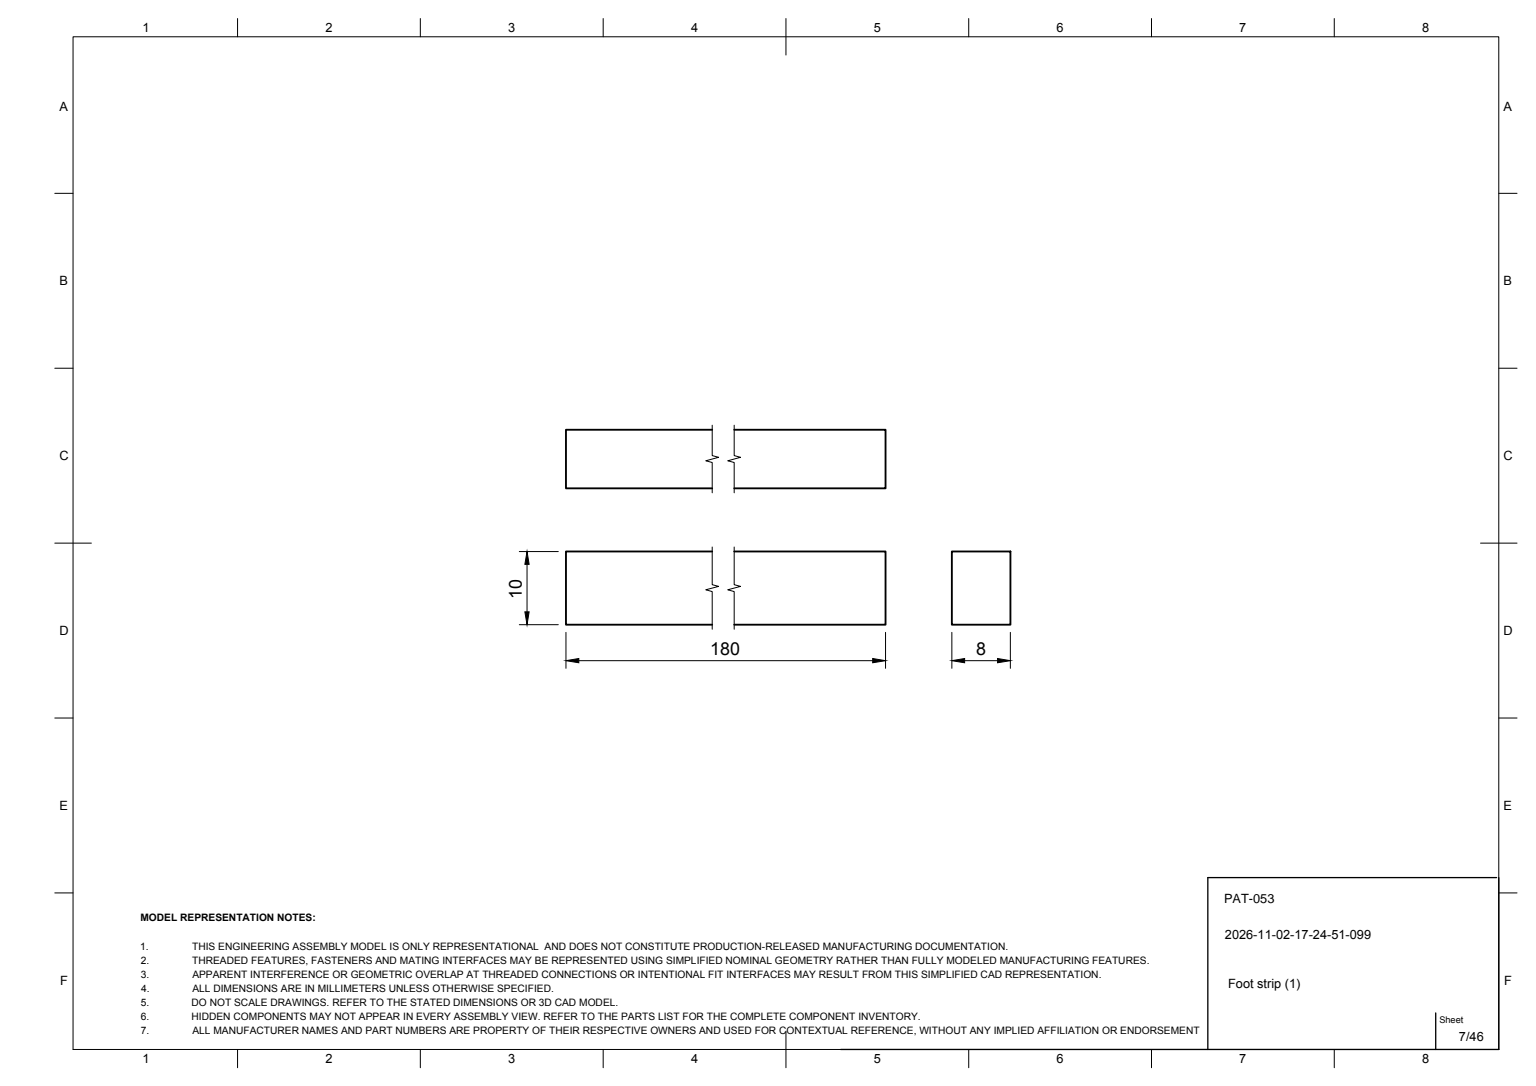
ISO-10303-21;
HEADER;
/* Generated by software containing ST-Developer
 * from STEP Tools, Inc. (www.steptools.com) 
 */

FILE_DESCRIPTION(
/* description */ ('Hand-operated arbor press'),
/* implementation_level */ '2;1');

FILE_NAME(
/* name */ 'Foot strip (1).step',
/* time_stamp */ '2026-10-28T03:25:25-07:00',
/* author */ (''),
/* organization */ (''),
/* preprocessor_version */ 'ST-DEVELOPER v20.2',
/* originating_system */ 'Autodesk Translation Framework v15.17.0.0',
/* authorisation */ '');

FILE_SCHEMA (('AUTOMOTIVE_DESIGN { 1 0 10303 214 3 1 1 }'));
ENDSEC;

DATA;
#10=MECHANICAL_DESIGN_GEOMETRIC_PRESENTATION_REPRESENTATION('',(#588),#32751);
#504=SHAPE_REPRESENTATION_RELATIONSHIP('SRR','None',#32933,#546);
#546=ADVANCED_BREP_SHAPE_REPRESENTATION('',(#637),#32707);
#588=STYLED_ITEM('',(#33228),#637);
#637=MANIFOLD_SOLID_BREP('Body1',#12485);
#861=PLANE('',#13046);
#862=PLANE('',#13047);
#863=PLANE('',#13048);
#864=PLANE('',#13049);
#865=PLANE('',#13050);
#866=PLANE('',#13051);
#1315=FACE_OUTER_BOUND('',#2016,.T.);
#1316=FACE_OUTER_BOUND('',#2017,.T.);
#1317=FACE_OUTER_BOUND('',#2018,.T.);
#1318=FACE_OUTER_BOUND('',#2019,.T.);
#1319=FACE_OUTER_BOUND('',#2020,.T.);
#1320=FACE_OUTER_BOUND('',#2021,.T.);
#2016=EDGE_LOOP('',(#8432,#8433,#8434,#8435));
#2017=EDGE_LOOP('',(#8436,#8437,#8438,#8439));
#2018=EDGE_LOOP('',(#8440,#8441,#8442,#8443));
#2019=EDGE_LOOP('',(#8444,#8445,#8446,#8447));
#2020=EDGE_LOOP('',(#8448,#8449,#8450,#8451));
#2021=EDGE_LOOP('',(#8452,#8453,#8454,#8455));
#2858=LINE('',#17758,#4029);
#2859=LINE('',#17760,#4030);
#2860=LINE('',#17762,#4031);
#2861=LINE('',#17763,#4032);
#2862=LINE('',#17766,#4033);
#2863=LINE('',#17768,#4034);
#2864=LINE('',#17769,#4035);
#2865=LINE('',#17772,#4036);
#2866=LINE('',#17774,#4037);
#2867=LINE('',#17775,#4038);
#2868=LINE('',#17777,#4039);
#2869=LINE('',#17778,#4040);
#4029=VECTOR('',#14285,1.);
#4030=VECTOR('',#14286,1.);
#4031=VECTOR('',#14287,1.);
#4032=VECTOR('',#14288,1.);
#4033=VECTOR('',#14291,1.);
#4034=VECTOR('',#14292,1.);
#4035=VECTOR('',#14293,1.);
#4036=VECTOR('',#14296,1.);
#4037=VECTOR('',#14297,1.);
#4038=VECTOR('',#14298,1.);
#4039=VECTOR('',#14301,1.);
#4040=VECTOR('',#14302,1.);
#5592=VERTEX_POINT('',#17756);
#5593=VERTEX_POINT('',#17757);
#5594=VERTEX_POINT('',#17759);
#5595=VERTEX_POINT('',#17761);
#5596=VERTEX_POINT('',#17765);
#5597=VERTEX_POINT('',#17767);
#5598=VERTEX_POINT('',#17771);
#5599=VERTEX_POINT('',#17773);
#6719=EDGE_CURVE('',#5592,#5593,#2858,.T.);
#6720=EDGE_CURVE('',#5593,#5594,#2859,.T.);
#6721=EDGE_CURVE('',#5595,#5594,#2860,.T.);
#6722=EDGE_CURVE('',#5592,#5595,#2861,.T.);
#6723=EDGE_CURVE('',#5596,#5592,#2862,.T.);
#6724=EDGE_CURVE('',#5597,#5595,#2863,.T.);
#6725=EDGE_CURVE('',#5596,#5597,#2864,.T.);
#6726=EDGE_CURVE('',#5598,#5596,#2865,.T.);
#6727=EDGE_CURVE('',#5599,#5597,#2866,.T.);
#6728=EDGE_CURVE('',#5598,#5599,#2867,.T.);
#6729=EDGE_CURVE('',#5593,#5598,#2868,.T.);
#6730=EDGE_CURVE('',#5594,#5599,#2869,.T.);
#8432=ORIENTED_EDGE('',*,*,#6719,.T.);
#8433=ORIENTED_EDGE('',*,*,#6720,.T.);
#8434=ORIENTED_EDGE('',*,*,#6721,.F.);
#8435=ORIENTED_EDGE('',*,*,#6722,.F.);
#8436=ORIENTED_EDGE('',*,*,#6723,.T.);
#8437=ORIENTED_EDGE('',*,*,#6722,.T.);
#8438=ORIENTED_EDGE('',*,*,#6724,.F.);
#8439=ORIENTED_EDGE('',*,*,#6725,.F.);
#8440=ORIENTED_EDGE('',*,*,#6726,.T.);
#8441=ORIENTED_EDGE('',*,*,#6725,.T.);
#8442=ORIENTED_EDGE('',*,*,#6727,.F.);
#8443=ORIENTED_EDGE('',*,*,#6728,.F.);
#8444=ORIENTED_EDGE('',*,*,#6729,.T.);
#8445=ORIENTED_EDGE('',*,*,#6728,.T.);
#8446=ORIENTED_EDGE('',*,*,#6730,.F.);
#8447=ORIENTED_EDGE('',*,*,#6720,.F.);
#8448=ORIENTED_EDGE('',*,*,#6730,.T.);
#8449=ORIENTED_EDGE('',*,*,#6727,.T.);
#8450=ORIENTED_EDGE('',*,*,#6724,.T.);
#8451=ORIENTED_EDGE('',*,*,#6721,.T.);
#8452=ORIENTED_EDGE('',*,*,#6729,.F.);
#8453=ORIENTED_EDGE('',*,*,#6719,.F.);
#8454=ORIENTED_EDGE('',*,*,#6723,.F.);
#8455=ORIENTED_EDGE('',*,*,#6726,.F.);
#11824=ADVANCED_FACE('',(#1315),#861,.T.);
#11825=ADVANCED_FACE('',(#1316),#862,.T.);
#11826=ADVANCED_FACE('',(#1317),#863,.T.);
#11827=ADVANCED_FACE('',(#1318),#864,.T.);
#11828=ADVANCED_FACE('',(#1319),#865,.T.);
#11829=ADVANCED_FACE('',(#1320),#866,.F.);
#12485=CLOSED_SHELL('',(#11824,#11825,#11826,#11827,#11828,#11829));
#13045=AXIS2_PLACEMENT_3D('',#17754,#14281,#14282);
#13046=AXIS2_PLACEMENT_3D('',#17755,#14283,#14284);
#13047=AXIS2_PLACEMENT_3D('',#17764,#14289,#14290);
#13048=AXIS2_PLACEMENT_3D('',#17770,#14294,#14295);
#13049=AXIS2_PLACEMENT_3D('',#17776,#14299,#14300);
#13050=AXIS2_PLACEMENT_3D('',#17779,#14303,#14304);
#13051=AXIS2_PLACEMENT_3D('',#17780,#14305,#14306);
#14281=DIRECTION('axis',(0.,0.,1.));
#14282=DIRECTION('refdir',(1.,0.,0.));
#14283=DIRECTION('center_axis',(0.,1.,0.));
#14284=DIRECTION('ref_axis',(-1.,0.,0.));
#14285=DIRECTION('',(-1.,0.,0.));
#14286=DIRECTION('',(0.,0.,1.));
#14287=DIRECTION('',(-1.,0.,0.));
#14288=DIRECTION('',(0.,0.,1.));
#14289=DIRECTION('center_axis',(1.,0.,0.));
#14290=DIRECTION('ref_axis',(0.,1.,0.));
#14291=DIRECTION('',(0.,1.,0.));
#14292=DIRECTION('',(0.,1.,0.));
#14293=DIRECTION('',(0.,0.,1.));
#14294=DIRECTION('center_axis',(0.,-1.,0.));
#14295=DIRECTION('ref_axis',(1.,0.,0.));
#14296=DIRECTION('',(1.,0.,0.));
#14297=DIRECTION('',(1.,0.,0.));
#14298=DIRECTION('',(0.,0.,1.));
#14299=DIRECTION('center_axis',(-1.,0.,0.));
#14300=DIRECTION('ref_axis',(0.,-1.,0.));
#14301=DIRECTION('',(0.,-1.,0.));
#14302=DIRECTION('',(0.,-1.,0.));
#14303=DIRECTION('center_axis',(0.,0.,1.));
#14304=DIRECTION('ref_axis',(1.,0.,0.));
#14305=DIRECTION('center_axis',(0.,0.,1.));
#14306=DIRECTION('ref_axis',(1.,0.,0.));
#17754=CARTESIAN_POINT('',(0.,0.,0.));
#17755=CARTESIAN_POINT('Origin',(10.,9.,-0.8));
#17756=CARTESIAN_POINT('',(10.,9.,-0.8));
#17757=CARTESIAN_POINT('',(9.,9.,-0.8));
#17758=CARTESIAN_POINT('',(10.,9.,-0.8));
#17759=CARTESIAN_POINT('',(9.,9.,0.));
#17760=CARTESIAN_POINT('',(9.,9.,-0.8));
#17761=CARTESIAN_POINT('',(10.,9.,0.));
#17762=CARTESIAN_POINT('',(10.,9.,0.));
#17763=CARTESIAN_POINT('',(10.,9.,-0.8));
#17764=CARTESIAN_POINT('Origin',(10.,-9.,-0.8));
#17765=CARTESIAN_POINT('',(10.,-9.,-0.8));
#17766=CARTESIAN_POINT('',(10.,-9.,-0.8));
#17767=CARTESIAN_POINT('',(10.,-9.,0.));
#17768=CARTESIAN_POINT('',(10.,-9.,0.));
#17769=CARTESIAN_POINT('',(10.,-9.,-0.8));
#17770=CARTESIAN_POINT('Origin',(9.,-9.,-0.8));
#17771=CARTESIAN_POINT('',(9.,-9.,-0.8));
#17772=CARTESIAN_POINT('',(9.,-9.,-0.8));
#17773=CARTESIAN_POINT('',(9.,-9.,0.));
#17774=CARTESIAN_POINT('',(9.,-9.,0.));
#17775=CARTESIAN_POINT('',(9.,-9.,-0.8));
#17776=CARTESIAN_POINT('Origin',(9.,9.,-0.8));
#17777=CARTESIAN_POINT('',(9.,9.,-0.8));
#17778=CARTESIAN_POINT('',(9.,9.,0.));
#17779=CARTESIAN_POINT('Origin',(9.5,0.,0.));
#17780=CARTESIAN_POINT('Origin',(9.5,0.,-0.8));
#32658=UNCERTAINTY_MEASURE_WITH_UNIT(LENGTH_MEASURE(0.001),#32752,
'DISTANCE_ACCURACY_VALUE',
'Maximum model space distance between geometric entities at asserted c
onnectivities');
#32702=UNCERTAINTY_MEASURE_WITH_UNIT(LENGTH_MEASURE(0.001),#32752,
'DISTANCE_ACCURACY_VALUE',
'Maximum model space distance between geometric entities at asserted c
onnectivities');
#32707=(
GEOMETRIC_REPRESENTATION_CONTEXT(3)
GLOBAL_UNCERTAINTY_ASSIGNED_CONTEXT((#32658))
GLOBAL_UNIT_ASSIGNED_CONTEXT((#32752,#32754,#32755))
REPRESENTATION_CONTEXT('','3D')
);
#32751=(
GEOMETRIC_REPRESENTATION_CONTEXT(3)
GLOBAL_UNCERTAINTY_ASSIGNED_CONTEXT((#32702))
GLOBAL_UNIT_ASSIGNED_CONTEXT((#32752,#32754,#32755))
REPRESENTATION_CONTEXT('','3D')
);
#32752=(
LENGTH_UNIT()
NAMED_UNIT(*)
SI_UNIT(.CENTI.,.METRE.)
);
#32754=(
NAMED_UNIT(*)
PLANE_ANGLE_UNIT()
SI_UNIT($,.RADIAN.)
);
#32755=(
NAMED_UNIT(*)
SI_UNIT($,.STERADIAN.)
SOLID_ANGLE_UNIT()
);
#32760=SHAPE_DEFINITION_REPRESENTATION(#32808,#32933);
#32808=PRODUCT_DEFINITION_SHAPE('',$,#32982);
#32933=SHAPE_REPRESENTATION('',(#13045),#32707);
#32977=PRODUCT_DEFINITION_CONTEXT('part definition',#33123,'design');
#32982=PRODUCT_DEFINITION('Foot strip (1)','Foot strip (1)',#33030,#32977);
#33030=PRODUCT_DEFINITION_FORMATION('',$,#33129);
#33123=APPLICATION_CONTEXT(
'Core Data for Automotive Mechanical Design Process');
#33124=PRODUCT_CONTEXT('part definition',#33123,'mechanical');
#33129=PRODUCT('Foot strip (1)','Foot strip (1)','Foot strip (1)',(#33124));
#33222=COLOUR_RGB('Light Blue',0.38,0.62,0.78);
#33223=FILL_AREA_STYLE_COLOUR('',#33222);
#33224=FILL_AREA_STYLE('',(#33223));
#33225=SURFACE_STYLE_FILL_AREA(#33224);
#33226=SURFACE_SIDE_STYLE('',(#33225));
#33227=SURFACE_STYLE_USAGE(.BOTH.,#33226);
#33228=PRESENTATION_STYLE_ASSIGNMENT((#33227));
ENDSEC;
END-ISO-10303-21;
